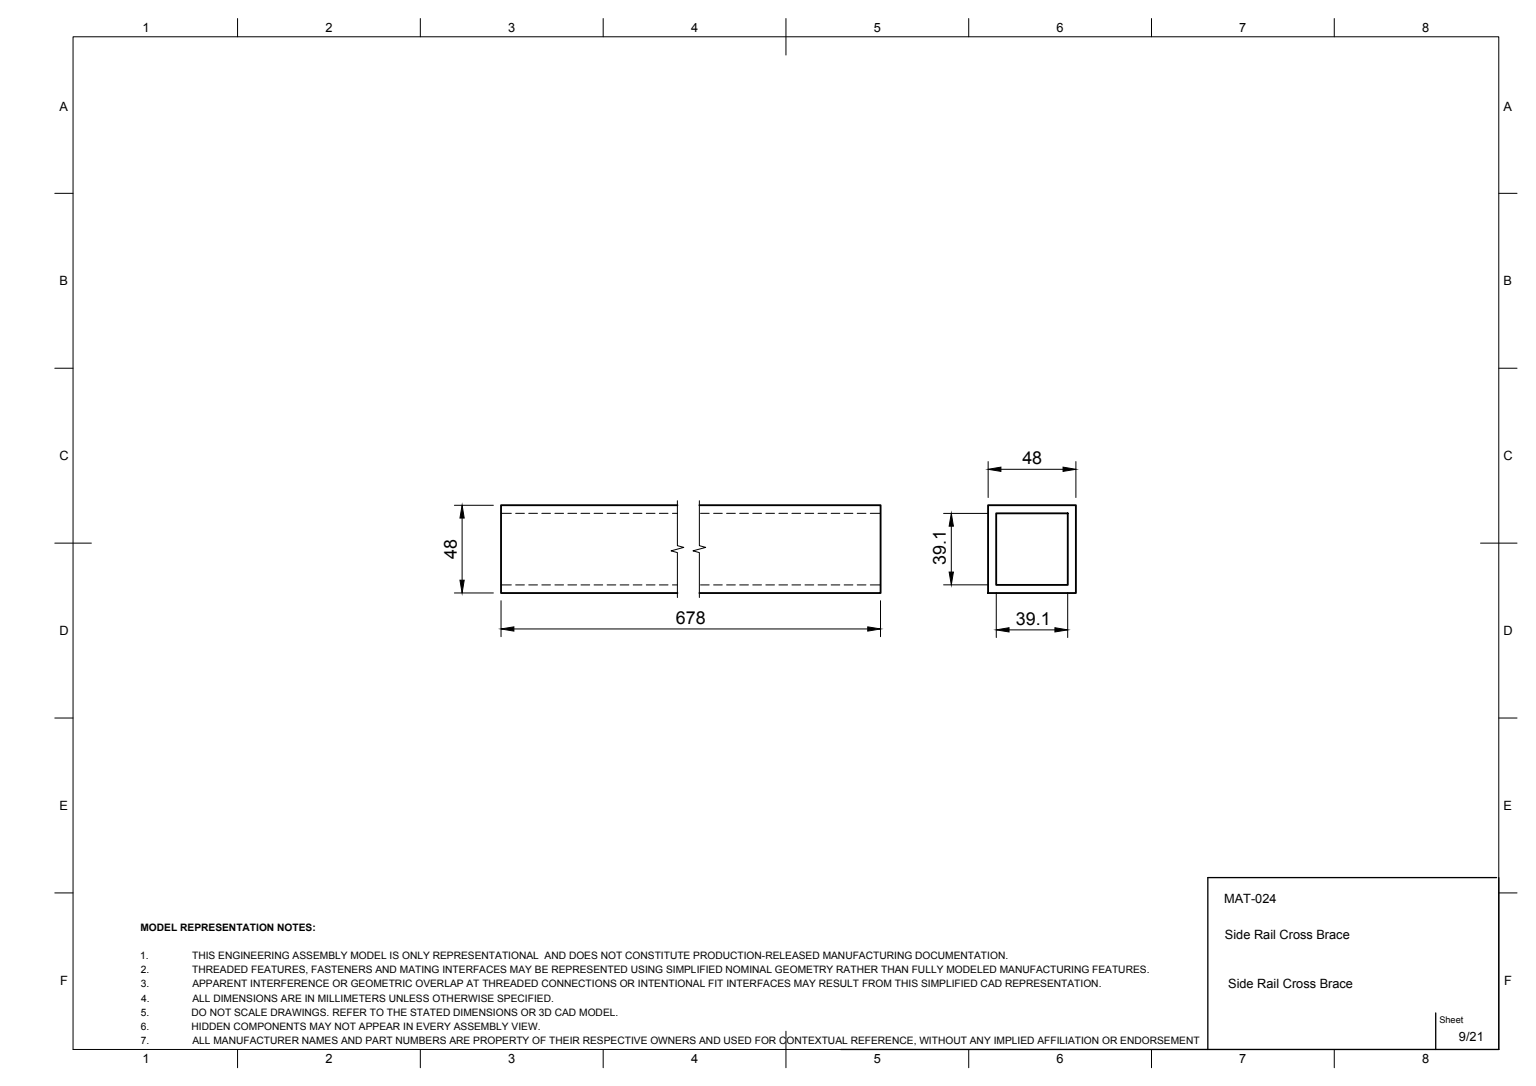
ISO-10303-21;
HEADER;
/* Generated by software containing ST-Developer
 * from STEP Tools, Inc. (www.steptools.com) 
 */

FILE_DESCRIPTION(
/* description */ ('STEP AP214'),
/* implementation_level */ '2;1');

FILE_NAME(
/* name */ 'Side Rail Cross Brace.step',
/* time_stamp */ '2026-11-14T06:34:07-08:00',
/* author */ (''),
/* organization */ (''),
/* preprocessor_version */ 'ST-DEVELOPER v20.2',
/* originating_system */ 'Autodesk Translation Framework v15.17.0.0',
/* authorisation */ '');

FILE_SCHEMA (('AUTOMOTIVE_DESIGN { 1 0 10303 214 3 1 1 }'));
ENDSEC;

DATA;
#10=MECHANICAL_DESIGN_GEOMETRIC_PRESENTATION_REPRESENTATION('',(#7318),#310623);
#7233=SHAPE_REPRESENTATION_RELATIONSHIP('SRR','None',#310906,#7250);
#7250=ADVANCED_BREP_SHAPE_REPRESENTATION('',(#7385),#310615);
#7318=STYLED_ITEM('',(#311004),#7385);
#7385=MANIFOLD_SOLID_BREP('Body1',#93769);
#7674=FACE_BOUND('',#20250,.T.);
#7675=FACE_BOUND('',#20252,.T.);
#8616=PLANE('',#104544);
#8617=PLANE('',#104545);
#8618=PLANE('',#104546);
#8619=PLANE('',#104547);
#8620=PLANE('',#104548);
#8621=PLANE('',#104549);
#8622=PLANE('',#104550);
#8623=PLANE('',#104551);
#8624=PLANE('',#104552);
#8625=PLANE('',#104553);
#14227=FACE_OUTER_BOUND('',#20249,.T.);
#14228=FACE_OUTER_BOUND('',#20251,.T.);
#14229=FACE_OUTER_BOUND('',#20253,.T.);
#14230=FACE_OUTER_BOUND('',#20254,.T.);
#14231=FACE_OUTER_BOUND('',#20255,.T.);
#14232=FACE_OUTER_BOUND('',#20256,.T.);
#14233=FACE_OUTER_BOUND('',#20257,.T.);
#14234=FACE_OUTER_BOUND('',#20258,.T.);
#14235=FACE_OUTER_BOUND('',#20259,.T.);
#14236=FACE_OUTER_BOUND('',#20260,.T.);
#20249=EDGE_LOOP('',(#84743,#84744,#84745,#84746));
#20250=EDGE_LOOP('',(#84747,#84748,#84749,#84750));
#20251=EDGE_LOOP('',(#84751,#84752,#84753,#84754));
#20252=EDGE_LOOP('',(#84755,#84756,#84757,#84758));
#20253=EDGE_LOOP('',(#84759,#84760,#84761,#84762));
#20254=EDGE_LOOP('',(#84763,#84764,#84765,#84766));
#20255=EDGE_LOOP('',(#84767,#84768,#84769,#84770));
#20256=EDGE_LOOP('',(#84771,#84772,#84773,#84774));
#20257=EDGE_LOOP('',(#84775,#84776,#84777,#84778));
#20258=EDGE_LOOP('',(#84779,#84780,#84781,#84782));
#20259=EDGE_LOOP('',(#84783,#84784,#84785,#84786));
#20260=EDGE_LOOP('',(#84787,#84788,#84789,#84790));
#24604=LINE('',#302736,#28951);
#24605=LINE('',#302738,#28952);
#24606=LINE('',#302740,#28953);
#24607=LINE('',#302741,#28954);
#24608=LINE('',#302744,#28955);
#24609=LINE('',#302746,#28956);
#24610=LINE('',#302748,#28957);
#24611=LINE('',#302749,#28958);
#24612=LINE('',#302753,#28959);
#24613=LINE('',#302755,#28960);
#24614=LINE('',#302757,#28961);
#24615=LINE('',#302758,#28962);
#24616=LINE('',#302761,#28963);
#24617=LINE('',#302763,#28964);
#24618=LINE('',#302765,#28965);
#24619=LINE('',#302766,#28966);
#24620=LINE('',#302768,#28967);
#24621=LINE('',#302769,#28968);
#24622=LINE('',#302771,#28969);
#24623=LINE('',#302773,#28970);
#24624=LINE('',#302776,#28971);
#24625=LINE('',#302777,#28972);
#24626=LINE('',#302779,#28973);
#24627=LINE('',#302781,#28974);
#28951=VECTOR('',#130151,1000.);
#28952=VECTOR('',#130152,1000.);
#28953=VECTOR('',#130153,1000.);
#28954=VECTOR('',#130154,1000.);
#28955=VECTOR('',#130155,1000.);
#28956=VECTOR('',#130156,1000.);
#28957=VECTOR('',#130157,1000.);
#28958=VECTOR('',#130158,1000.);
#28959=VECTOR('',#130161,1000.);
#28960=VECTOR('',#130162,1000.);
#28961=VECTOR('',#130163,1000.);
#28962=VECTOR('',#130164,1000.);
#28963=VECTOR('',#130165,1000.);
#28964=VECTOR('',#130166,1000.);
#28965=VECTOR('',#130167,1000.);
#28966=VECTOR('',#130168,1000.);
#28967=VECTOR('',#130171,1000.);
#28968=VECTOR('',#130172,1000.);
#28969=VECTOR('',#130175,1000.);
#28970=VECTOR('',#130178,1000.);
#28971=VECTOR('',#130183,1000.);
#28972=VECTOR('',#130184,1000.);
#28973=VECTOR('',#130187,1000.);
#28974=VECTOR('',#130190,1000.);
#43282=VERTEX_POINT('',#302734);
#43283=VERTEX_POINT('',#302735);
#43284=VERTEX_POINT('',#302737);
#43285=VERTEX_POINT('',#302739);
#43286=VERTEX_POINT('',#302742);
#43287=VERTEX_POINT('',#302743);
#43288=VERTEX_POINT('',#302745);
#43289=VERTEX_POINT('',#302747);
#43290=VERTEX_POINT('',#302751);
#43291=VERTEX_POINT('',#302752);
#43292=VERTEX_POINT('',#302754);
#43293=VERTEX_POINT('',#302756);
#43294=VERTEX_POINT('',#302759);
#43295=VERTEX_POINT('',#302760);
#43296=VERTEX_POINT('',#302762);
#43297=VERTEX_POINT('',#302764);
#57151=EDGE_CURVE('',#43282,#43283,#24604,.T.);
#57152=EDGE_CURVE('',#43283,#43284,#24605,.T.);
#57153=EDGE_CURVE('',#43284,#43285,#24606,.T.);
#57154=EDGE_CURVE('',#43285,#43282,#24607,.T.);
#57155=EDGE_CURVE('',#43286,#43287,#24608,.T.);
#57156=EDGE_CURVE('',#43288,#43286,#24609,.T.);
#57157=EDGE_CURVE('',#43289,#43288,#24610,.T.);
#57158=EDGE_CURVE('',#43287,#43289,#24611,.T.);
#57159=EDGE_CURVE('',#43290,#43291,#24612,.T.);
#57160=EDGE_CURVE('',#43292,#43290,#24613,.T.);
#57161=EDGE_CURVE('',#43293,#43292,#24614,.T.);
#57162=EDGE_CURVE('',#43291,#43293,#24615,.T.);
#57163=EDGE_CURVE('',#43294,#43295,#24616,.T.);
#57164=EDGE_CURVE('',#43295,#43296,#24617,.T.);
#57165=EDGE_CURVE('',#43296,#43297,#24618,.T.);
#57166=EDGE_CURVE('',#43297,#43294,#24619,.T.);
#57167=EDGE_CURVE('',#43283,#43291,#24620,.T.);
#57168=EDGE_CURVE('',#43282,#43290,#24621,.T.);
#57169=EDGE_CURVE('',#43284,#43293,#24622,.T.);
#57170=EDGE_CURVE('',#43285,#43292,#24623,.T.);
#57171=EDGE_CURVE('',#43286,#43295,#24624,.T.);
#57172=EDGE_CURVE('',#43287,#43296,#24625,.T.);
#57173=EDGE_CURVE('',#43289,#43297,#24626,.T.);
#57174=EDGE_CURVE('',#43288,#43294,#24627,.T.);
#84743=ORIENTED_EDGE('',*,*,#57151,.T.);
#84744=ORIENTED_EDGE('',*,*,#57152,.T.);
#84745=ORIENTED_EDGE('',*,*,#57153,.T.);
#84746=ORIENTED_EDGE('',*,*,#57154,.T.);
#84747=ORIENTED_EDGE('',*,*,#57155,.F.);
#84748=ORIENTED_EDGE('',*,*,#57156,.F.);
#84749=ORIENTED_EDGE('',*,*,#57157,.F.);
#84750=ORIENTED_EDGE('',*,*,#57158,.F.);
#84751=ORIENTED_EDGE('',*,*,#57159,.F.);
#84752=ORIENTED_EDGE('',*,*,#57160,.F.);
#84753=ORIENTED_EDGE('',*,*,#57161,.F.);
#84754=ORIENTED_EDGE('',*,*,#57162,.F.);
#84755=ORIENTED_EDGE('',*,*,#57163,.T.);
#84756=ORIENTED_EDGE('',*,*,#57164,.T.);
#84757=ORIENTED_EDGE('',*,*,#57165,.T.);
#84758=ORIENTED_EDGE('',*,*,#57166,.T.);
#84759=ORIENTED_EDGE('',*,*,#57159,.T.);
#84760=ORIENTED_EDGE('',*,*,#57167,.F.);
#84761=ORIENTED_EDGE('',*,*,#57151,.F.);
#84762=ORIENTED_EDGE('',*,*,#57168,.T.);
#84763=ORIENTED_EDGE('',*,*,#57162,.T.);
#84764=ORIENTED_EDGE('',*,*,#57169,.F.);
#84765=ORIENTED_EDGE('',*,*,#57152,.F.);
#84766=ORIENTED_EDGE('',*,*,#57167,.T.);
#84767=ORIENTED_EDGE('',*,*,#57161,.T.);
#84768=ORIENTED_EDGE('',*,*,#57170,.F.);
#84769=ORIENTED_EDGE('',*,*,#57153,.F.);
#84770=ORIENTED_EDGE('',*,*,#57169,.T.);
#84771=ORIENTED_EDGE('',*,*,#57160,.T.);
#84772=ORIENTED_EDGE('',*,*,#57168,.F.);
#84773=ORIENTED_EDGE('',*,*,#57154,.F.);
#84774=ORIENTED_EDGE('',*,*,#57170,.T.);
#84775=ORIENTED_EDGE('',*,*,#57164,.F.);
#84776=ORIENTED_EDGE('',*,*,#57171,.F.);
#84777=ORIENTED_EDGE('',*,*,#57155,.T.);
#84778=ORIENTED_EDGE('',*,*,#57172,.T.);
#84779=ORIENTED_EDGE('',*,*,#57165,.F.);
#84780=ORIENTED_EDGE('',*,*,#57172,.F.);
#84781=ORIENTED_EDGE('',*,*,#57158,.T.);
#84782=ORIENTED_EDGE('',*,*,#57173,.T.);
#84783=ORIENTED_EDGE('',*,*,#57166,.F.);
#84784=ORIENTED_EDGE('',*,*,#57173,.F.);
#84785=ORIENTED_EDGE('',*,*,#57157,.T.);
#84786=ORIENTED_EDGE('',*,*,#57174,.T.);
#84787=ORIENTED_EDGE('',*,*,#57163,.F.);
#84788=ORIENTED_EDGE('',*,*,#57174,.F.);
#84789=ORIENTED_EDGE('',*,*,#57156,.T.);
#84790=ORIENTED_EDGE('',*,*,#57171,.T.);
#93506=ADVANCED_FACE('',(#14227,#7674),#8616,.F.);
#93507=ADVANCED_FACE('',(#14228,#7675),#8617,.T.);
#93508=ADVANCED_FACE('',(#14229),#8618,.F.);
#93509=ADVANCED_FACE('',(#14230),#8619,.F.);
#93510=ADVANCED_FACE('',(#14231),#8620,.F.);
#93511=ADVANCED_FACE('',(#14232),#8621,.F.);
#93512=ADVANCED_FACE('',(#14233),#8622,.T.);
#93513=ADVANCED_FACE('',(#14234),#8623,.T.);
#93514=ADVANCED_FACE('',(#14235),#8624,.T.);
#93515=ADVANCED_FACE('',(#14236),#8625,.T.);
#93769=CLOSED_SHELL('',(#93506,#93507,#93508,#93509,#93510,#93511,#93512,
#93513,#93514,#93515));
#104543=AXIS2_PLACEMENT_3D('',#302732,#130147,#130148);
#104544=AXIS2_PLACEMENT_3D('',#302733,#130149,#130150);
#104545=AXIS2_PLACEMENT_3D('',#302750,#130159,#130160);
#104546=AXIS2_PLACEMENT_3D('',#302767,#130169,#130170);
#104547=AXIS2_PLACEMENT_3D('',#302770,#130173,#130174);
#104548=AXIS2_PLACEMENT_3D('',#302772,#130176,#130177);
#104549=AXIS2_PLACEMENT_3D('',#302774,#130179,#130180);
#104550=AXIS2_PLACEMENT_3D('',#302775,#130181,#130182);
#104551=AXIS2_PLACEMENT_3D('',#302778,#130185,#130186);
#104552=AXIS2_PLACEMENT_3D('',#302780,#130188,#130189);
#104553=AXIS2_PLACEMENT_3D('',#302782,#130191,#130192);
#130147=DIRECTION('axis',(0.,0.,1.));
#130148=DIRECTION('refdir',(1.,0.,0.));
#130149=DIRECTION('center_axis',(0.,0.,-1.));
#130150=DIRECTION('ref_axis',(-1.,0.,0.));
#130151=DIRECTION('',(0.,1.,0.));
#130152=DIRECTION('',(-1.,0.,0.));
#130153=DIRECTION('',(0.,-1.,0.));
#130154=DIRECTION('',(1.,0.,0.));
#130155=DIRECTION('',(0.,1.,0.));
#130156=DIRECTION('',(1.,0.,0.));
#130157=DIRECTION('',(0.,-1.,0.));
#130158=DIRECTION('',(-1.,0.,0.));
#130159=DIRECTION('center_axis',(0.,0.,-1.));
#130160=DIRECTION('ref_axis',(-1.,0.,0.));
#130161=DIRECTION('',(0.,1.,0.));
#130162=DIRECTION('',(1.,0.,0.));
#130163=DIRECTION('',(0.,-1.,0.));
#130164=DIRECTION('',(-1.,0.,0.));
#130165=DIRECTION('',(1.,0.,0.));
#130166=DIRECTION('',(0.,1.,0.));
#130167=DIRECTION('',(-1.,0.,0.));
#130168=DIRECTION('',(0.,-1.,0.));
#130169=DIRECTION('center_axis',(-1.,0.,0.));
#130170=DIRECTION('ref_axis',(0.,0.,1.));
#130171=DIRECTION('',(0.,0.,-1.));
#130172=DIRECTION('',(0.,0.,-1.));
#130173=DIRECTION('center_axis',(0.,-1.,0.));
#130174=DIRECTION('ref_axis',(0.,0.,-1.));
#130175=DIRECTION('',(0.,0.,-1.));
#130176=DIRECTION('center_axis',(1.,0.,0.));
#130177=DIRECTION('ref_axis',(0.,0.,-1.));
#130178=DIRECTION('',(0.,0.,-1.));
#130179=DIRECTION('center_axis',(0.,1.,0.));
#130180=DIRECTION('ref_axis',(0.,0.,1.));
#130181=DIRECTION('center_axis',(-1.,0.,0.));
#130182=DIRECTION('ref_axis',(0.,0.,1.));
#130183=DIRECTION('',(0.,0.,-1.));
#130184=DIRECTION('',(0.,0.,-1.));
#130185=DIRECTION('center_axis',(0.,-1.,0.));
#130186=DIRECTION('ref_axis',(0.,0.,-1.));
#130187=DIRECTION('',(0.,0.,-1.));
#130188=DIRECTION('center_axis',(1.,0.,0.));
#130189=DIRECTION('ref_axis',(0.,0.,-1.));
#130190=DIRECTION('',(0.,0.,-1.));
#130191=DIRECTION('center_axis',(0.,1.,0.));
#130192=DIRECTION('ref_axis',(0.,0.,1.));
#302732=CARTESIAN_POINT('',(0.,0.,0.));
#302733=CARTESIAN_POINT('Origin',(0.,0.,678.));
#302734=CARTESIAN_POINT('',(24.,-24.,678.));
#302735=CARTESIAN_POINT('',(24.,24.,678.));
#302736=CARTESIAN_POINT('',(24.,-24.,678.));
#302737=CARTESIAN_POINT('',(-24.,24.,678.));
#302738=CARTESIAN_POINT('',(-24.,24.,678.));
#302739=CARTESIAN_POINT('',(-24.,-24.,678.));
#302740=CARTESIAN_POINT('',(-24.,-24.,678.));
#302741=CARTESIAN_POINT('',(-24.,-24.,678.));
#302742=CARTESIAN_POINT('',(19.55,-19.55,678.));
#302743=CARTESIAN_POINT('',(19.55,19.55,678.));
#302744=CARTESIAN_POINT('',(19.55,-19.55,678.));
#302745=CARTESIAN_POINT('',(-19.55,-19.55,678.));
#302746=CARTESIAN_POINT('',(-19.55,-19.55,678.));
#302747=CARTESIAN_POINT('',(-19.55,19.55,678.));
#302748=CARTESIAN_POINT('',(-19.55,-19.55,678.));
#302749=CARTESIAN_POINT('',(-19.55,19.55,678.));
#302750=CARTESIAN_POINT('Origin',(0.,0.,0.));
#302751=CARTESIAN_POINT('',(24.,-24.,0.));
#302752=CARTESIAN_POINT('',(24.,24.,0.));
#302753=CARTESIAN_POINT('',(24.,-24.,0.));
#302754=CARTESIAN_POINT('',(-24.,-24.,0.));
#302755=CARTESIAN_POINT('',(-24.,-24.,0.));
#302756=CARTESIAN_POINT('',(-24.,24.,0.));
#302757=CARTESIAN_POINT('',(-24.,-24.,0.));
#302758=CARTESIAN_POINT('',(-24.,24.,0.));
#302759=CARTESIAN_POINT('',(-19.55,-19.55,0.));
#302760=CARTESIAN_POINT('',(19.55,-19.55,0.));
#302761=CARTESIAN_POINT('',(-19.55,-19.55,0.));
#302762=CARTESIAN_POINT('',(19.55,19.55,0.));
#302763=CARTESIAN_POINT('',(19.55,-19.55,0.));
#302764=CARTESIAN_POINT('',(-19.55,19.55,0.));
#302765=CARTESIAN_POINT('',(-19.55,19.55,0.));
#302766=CARTESIAN_POINT('',(-19.55,-19.55,0.));
#302767=CARTESIAN_POINT('Origin',(24.,-24.,678.));
#302768=CARTESIAN_POINT('',(24.,24.,678.));
#302769=CARTESIAN_POINT('',(24.,-24.,678.));
#302770=CARTESIAN_POINT('Origin',(-24.,24.,678.));
#302771=CARTESIAN_POINT('',(-24.,24.,678.));
#302772=CARTESIAN_POINT('Origin',(-24.,-24.,678.));
#302773=CARTESIAN_POINT('',(-24.,-24.,678.));
#302774=CARTESIAN_POINT('Origin',(-24.,-24.,678.));
#302775=CARTESIAN_POINT('Origin',(19.55,-19.55,678.));
#302776=CARTESIAN_POINT('',(19.55,-19.55,678.));
#302777=CARTESIAN_POINT('',(19.55,19.55,678.));
#302778=CARTESIAN_POINT('Origin',(-19.55,19.55,678.));
#302779=CARTESIAN_POINT('',(-19.55,19.55,678.));
#302780=CARTESIAN_POINT('Origin',(-19.55,-19.55,678.));
#302781=CARTESIAN_POINT('',(-19.55,-19.55,678.));
#302782=CARTESIAN_POINT('Origin',(-19.55,-19.55,678.));
#310593=UNCERTAINTY_MEASURE_WITH_UNIT(LENGTH_MEASURE(0.01),#310624,
'DISTANCE_ACCURACY_VALUE',
'Maximum model space distance between geometric entities at asserted c
onnectivities');
#310601=UNCERTAINTY_MEASURE_WITH_UNIT(LENGTH_MEASURE(0.01),#310624,
'DISTANCE_ACCURACY_VALUE',
'Maximum model space distance between geometric entities at asserted c
onnectivities');
#310615=(
GEOMETRIC_REPRESENTATION_CONTEXT(3)
GLOBAL_UNCERTAINTY_ASSIGNED_CONTEXT((#310593))
GLOBAL_UNIT_ASSIGNED_CONTEXT((#310624,#310626,#310627))
REPRESENTATION_CONTEXT('','3D')
);
#310623=(
GEOMETRIC_REPRESENTATION_CONTEXT(3)
GLOBAL_UNCERTAINTY_ASSIGNED_CONTEXT((#310601))
GLOBAL_UNIT_ASSIGNED_CONTEXT((#310624,#310626,#310627))
REPRESENTATION_CONTEXT('','3D')
);
#310624=(
LENGTH_UNIT()
NAMED_UNIT(*)
SI_UNIT(.MILLI.,.METRE.)
);
#310626=(
NAMED_UNIT(*)
PLANE_ANGLE_UNIT()
SI_UNIT($,.RADIAN.)
);
#310627=(
NAMED_UNIT(*)
SI_UNIT($,.STERADIAN.)
SOLID_ANGLE_UNIT()
);
#310641=SHAPE_DEFINITION_REPRESENTATION(#310800,#310906);
#310800=PRODUCT_DEFINITION_SHAPE('',$,#310928);
#310906=SHAPE_REPRESENTATION('',(#104543),#310615);
#310914=PRODUCT_DEFINITION_CONTEXT('part definition',#310979,'design');
#310928=PRODUCT_DEFINITION('Side Rail Cross Brace',
'Side Rail Cross Brace',#310949,#310914);
#310949=PRODUCT_DEFINITION_FORMATION('',$,#310994);
#310979=APPLICATION_CONTEXT(
'Core Data for Automotive Mechanical Design Process');
#310980=PRODUCT_CONTEXT('part definition',#310979,'mechanical');
#310994=PRODUCT('Side Rail Cross Brace','Side Rail Cross Brace',$,(#310980));
#311004=PRESENTATION_STYLE_ASSIGNMENT((#311011));
#311011=SURFACE_STYLE_USAGE(.BOTH.,#311018);
#311018=SURFACE_SIDE_STYLE('',(#311025));
#311025=SURFACE_STYLE_FILL_AREA(#311032);
#311032=FILL_AREA_STYLE('Opaque(227,224,212)',(#311039));
#311039=FILL_AREA_STYLE_COLOUR('Opaque(227,224,212)',#311046);
#311046=COLOUR_RGB('Opaque(227,224,212)',0.890196078431372,0.87843137254902,
0.831372549019608);
ENDSEC;
END-ISO-10303-21;
